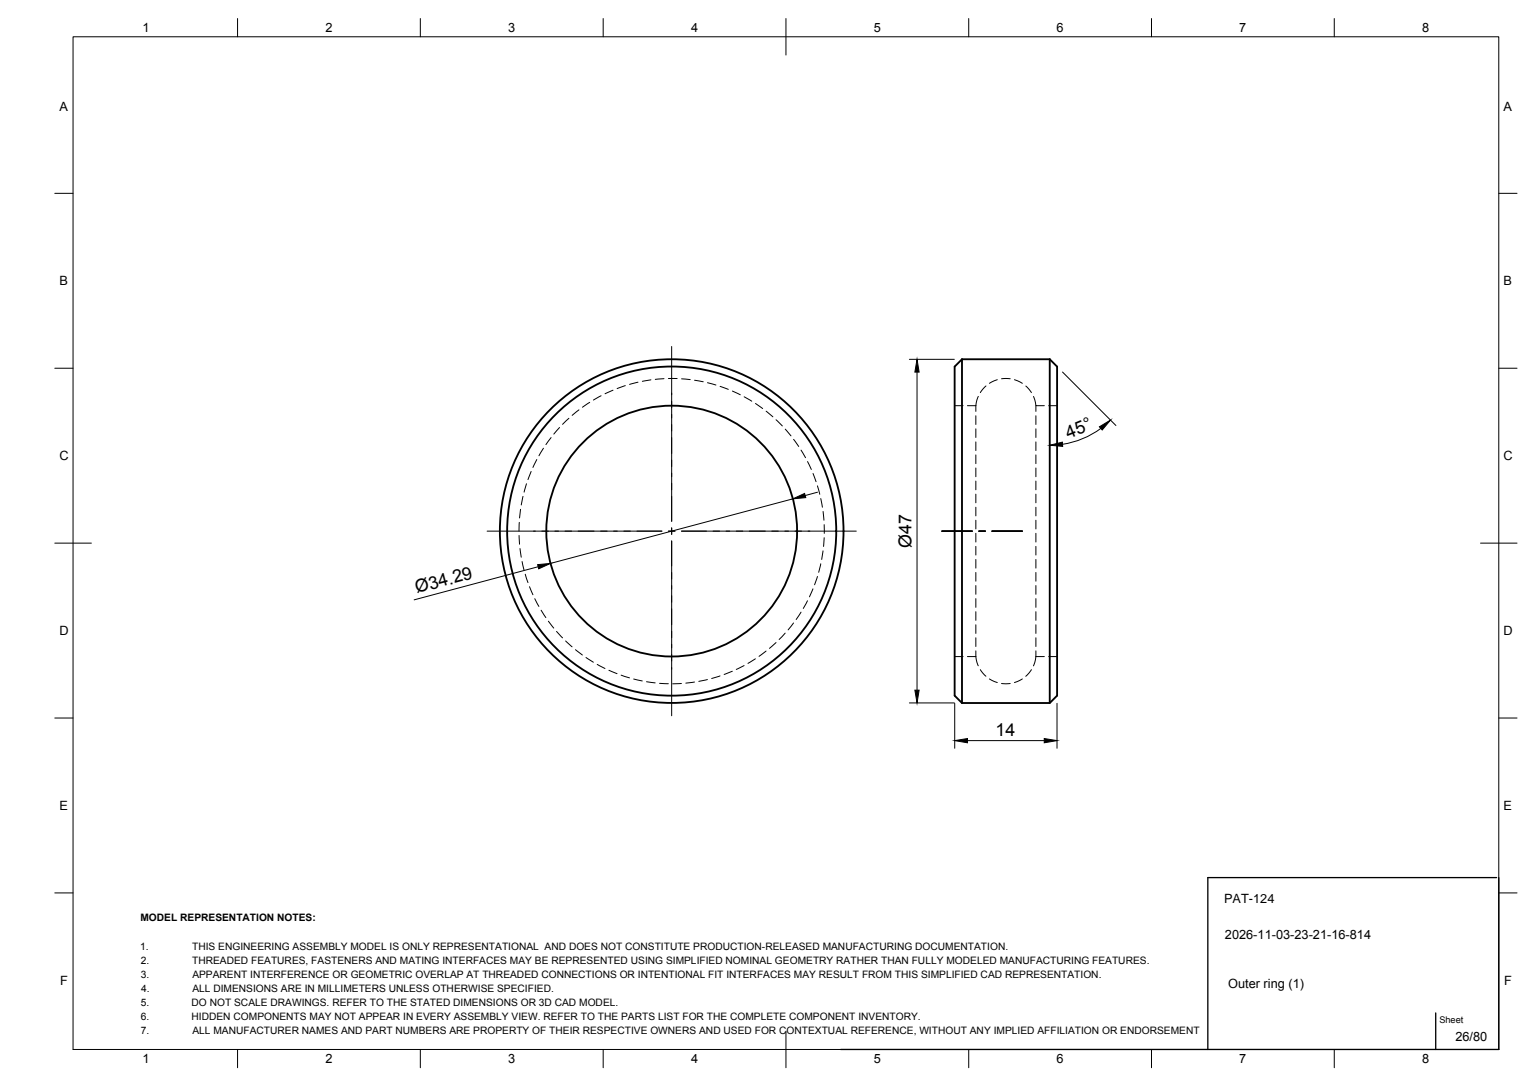
ISO-10303-21;
HEADER;
/* Generated by software containing ST-Developer
 * from STEP Tools, Inc. (www.steptools.com) 
 */

FILE_DESCRIPTION(
/* description */ ('XY cross-slide table'),
/* implementation_level */ '2;1');

FILE_NAME(
/* name */ 'Outer ring (1).step',
/* time_stamp */ '2026-10-28T03:22:46-07:00',
/* author */ (''),
/* organization */ (''),
/* preprocessor_version */ 'ST-DEVELOPER v20.2',
/* originating_system */ 'Autodesk Translation Framework v15.17.0.0',
/* authorisation */ '');

FILE_SCHEMA (('AUTOMOTIVE_DESIGN { 1 0 10303 214 3 1 1 }'));
ENDSEC;

DATA;
#10=MECHANICAL_DESIGN_GEOMETRIC_PRESENTATION_REPRESENTATION('',(#1694),#62984);
#1447=CONICAL_SURFACE('',#24446,2.3,0.785398163397449);
#1448=CONICAL_SURFACE('',#24450,2.3,0.785398163397449);
#1499=TOROIDAL_SURFACE('',#24435,1.675,0.412776);
#1521=SHAPE_REPRESENTATION_RELATIONSHIP('SRR','None',#63371,#1604);
#1604=ADVANCED_BREP_SHAPE_REPRESENTATION('',(#1807),#62908);
#1694=STYLED_ITEM('',(#63912),#1807);
#1807=MANIFOLD_SOLID_BREP('Body1',#22988);
#1994=FACE_BOUND('',#4496,.T.);
#1995=FACE_BOUND('',#4501,.T.);
#2399=PLANE('',#24443);
#2400=PLANE('',#24452);
#3072=FACE_OUTER_BOUND('',#4493,.T.);
#3073=FACE_OUTER_BOUND('',#4494,.T.);
#3074=FACE_OUTER_BOUND('',#4495,.T.);
#3075=FACE_OUTER_BOUND('',#4497,.T.);
#3076=FACE_OUTER_BOUND('',#4498,.T.);
#3077=FACE_OUTER_BOUND('',#4499,.T.);
#3078=FACE_OUTER_BOUND('',#4500,.T.);
#3079=FACE_OUTER_BOUND('',#4502,.T.);
#4493=EDGE_LOOP('',(#15784,#15785,#15786,#15787,#15788,#15789));
#4494=EDGE_LOOP('',(#15790,#15791,#15792,#15793,#15794));
#4495=EDGE_LOOP('',(#15795));
#4496=EDGE_LOOP('',(#15796));
#4497=EDGE_LOOP('',(#15797,#15798,#15799,#15800));
#4498=EDGE_LOOP('',(#15801,#15802,#15803,#15804));
#4499=EDGE_LOOP('',(#15805,#15806,#15807,#15808));
#4500=EDGE_LOOP('',(#15809));
#4501=EDGE_LOOP('',(#15810));
#4502=EDGE_LOOP('',(#15811,#15812,#15813,#15814,#15815));
#6128=LINE('',#34146,#7615);
#6129=LINE('',#34155,#7616);
#6130=LINE('',#34159,#7617);
#6131=LINE('',#34163,#7618);
#6132=LINE('',#34166,#7619);
#7615=VECTOR('',#27569,1.71469);
#7616=VECTOR('',#27580,2.3);
#7617=VECTOR('',#27585,2.35);
#7618=VECTOR('',#27590,2.3);
#7619=VECTOR('',#27595,1.71469);
#9084=CIRCLE('',#24436,1.71469);
#9085=CIRCLE('',#24437,1.71469);
#9086=CIRCLE('',#24438,0.412776);
#9087=CIRCLE('',#24439,1.71469);
#9088=CIRCLE('',#24440,1.71469);
#9089=CIRCLE('',#24442,1.71469);
#9090=CIRCLE('',#24444,2.25);
#9091=CIRCLE('',#24445,1.71469);
#9092=CIRCLE('',#24447,2.35);
#9093=CIRCLE('',#24449,2.35);
#9094=CIRCLE('',#24451,2.25);
#10071=VERTEX_POINT('',#34134);
#10072=VERTEX_POINT('',#34135);
#10073=VERTEX_POINT('',#34138);
#10074=VERTEX_POINT('',#34140);
#10075=VERTEX_POINT('',#34144);
#10076=VERTEX_POINT('',#34148);
#10077=VERTEX_POINT('',#34150);
#10078=VERTEX_POINT('',#34153);
#10079=VERTEX_POINT('',#34157);
#10080=VERTEX_POINT('',#34161);
#12276=EDGE_CURVE('',#10071,#10072,#9084,.T.);
#12277=EDGE_CURVE('',#10072,#10071,#9085,.T.);
#12278=EDGE_CURVE('',#10072,#10073,#9086,.T.);
#12279=EDGE_CURVE('',#10074,#10073,#9087,.T.);
#12280=EDGE_CURVE('',#10073,#10074,#9088,.T.);
#12281=EDGE_CURVE('',#10075,#10075,#9089,.T.);
#12282=EDGE_CURVE('',#10075,#10074,#6128,.T.);
#12283=EDGE_CURVE('',#10076,#10076,#9090,.T.);
#12284=EDGE_CURVE('',#10077,#10077,#9091,.T.);
#12285=EDGE_CURVE('',#10078,#10078,#9092,.T.);
#12286=EDGE_CURVE('',#10078,#10076,#6129,.T.);
#12287=EDGE_CURVE('',#10079,#10079,#9093,.T.);
#12288=EDGE_CURVE('',#10079,#10078,#6130,.T.);
#12289=EDGE_CURVE('',#10080,#10080,#9094,.T.);
#12290=EDGE_CURVE('',#10080,#10079,#6131,.T.);
#12291=EDGE_CURVE('',#10071,#10077,#6132,.T.);
#15784=ORIENTED_EDGE('',*,*,#12276,.F.);
#15785=ORIENTED_EDGE('',*,*,#12277,.F.);
#15786=ORIENTED_EDGE('',*,*,#12278,.T.);
#15787=ORIENTED_EDGE('',*,*,#12279,.F.);
#15788=ORIENTED_EDGE('',*,*,#12280,.F.);
#15789=ORIENTED_EDGE('',*,*,#12278,.F.);
#15790=ORIENTED_EDGE('',*,*,#12281,.T.);
#15791=ORIENTED_EDGE('',*,*,#12282,.T.);
#15792=ORIENTED_EDGE('',*,*,#12279,.T.);
#15793=ORIENTED_EDGE('',*,*,#12280,.T.);
#15794=ORIENTED_EDGE('',*,*,#12282,.F.);
#15795=ORIENTED_EDGE('',*,*,#12283,.F.);
#15796=ORIENTED_EDGE('',*,*,#12284,.T.);
#15797=ORIENTED_EDGE('',*,*,#12285,.F.);
#15798=ORIENTED_EDGE('',*,*,#12286,.T.);
#15799=ORIENTED_EDGE('',*,*,#12283,.T.);
#15800=ORIENTED_EDGE('',*,*,#12286,.F.);
#15801=ORIENTED_EDGE('',*,*,#12287,.F.);
#15802=ORIENTED_EDGE('',*,*,#12288,.T.);
#15803=ORIENTED_EDGE('',*,*,#12285,.T.);
#15804=ORIENTED_EDGE('',*,*,#12288,.F.);
#15805=ORIENTED_EDGE('',*,*,#12289,.F.);
#15806=ORIENTED_EDGE('',*,*,#12290,.T.);
#15807=ORIENTED_EDGE('',*,*,#12287,.T.);
#15808=ORIENTED_EDGE('',*,*,#12290,.F.);
#15809=ORIENTED_EDGE('',*,*,#12289,.T.);
#15810=ORIENTED_EDGE('',*,*,#12281,.F.);
#15811=ORIENTED_EDGE('',*,*,#12276,.T.);
#15812=ORIENTED_EDGE('',*,*,#12277,.T.);
#15813=ORIENTED_EDGE('',*,*,#12291,.T.);
#15814=ORIENTED_EDGE('',*,*,#12284,.F.);
#15815=ORIENTED_EDGE('',*,*,#12291,.F.);
#21117=CYLINDRICAL_SURFACE('',#24441,1.71469);
#21118=CYLINDRICAL_SURFACE('',#24448,2.35);
#21119=CYLINDRICAL_SURFACE('',#24453,1.71469);
#21853=ADVANCED_FACE('',(#3072),#1499,.F.);
#21854=ADVANCED_FACE('',(#3073),#21117,.F.);
#21855=ADVANCED_FACE('',(#3074,#1994),#2399,.T.);
#21856=ADVANCED_FACE('',(#3075),#1447,.T.);
#21857=ADVANCED_FACE('',(#3076),#21118,.T.);
#21858=ADVANCED_FACE('',(#3077),#1448,.T.);
#21859=ADVANCED_FACE('',(#3078,#1995),#2400,.T.);
#21860=ADVANCED_FACE('',(#3079),#21119,.F.);
#22988=CLOSED_SHELL('',(#21853,#21854,#21855,#21856,#21857,#21858,#21859,
#21860));
#24434=AXIS2_PLACEMENT_3D('',#34132,#27551,#27552);
#24435=AXIS2_PLACEMENT_3D('',#34133,#27553,#27554);
#24436=AXIS2_PLACEMENT_3D('',#34136,#27555,#27556);
#24437=AXIS2_PLACEMENT_3D('',#34137,#27557,#27558);
#24438=AXIS2_PLACEMENT_3D('',#34139,#27559,#27560);
#24439=AXIS2_PLACEMENT_3D('',#34141,#27561,#27562);
#24440=AXIS2_PLACEMENT_3D('',#34142,#27563,#27564);
#24441=AXIS2_PLACEMENT_3D('',#34143,#27565,#27566);
#24442=AXIS2_PLACEMENT_3D('',#34145,#27567,#27568);
#24443=AXIS2_PLACEMENT_3D('',#34147,#27570,#27571);
#24444=AXIS2_PLACEMENT_3D('',#34149,#27572,#27573);
#24445=AXIS2_PLACEMENT_3D('',#34151,#27574,#27575);
#24446=AXIS2_PLACEMENT_3D('',#34152,#27576,#27577);
#24447=AXIS2_PLACEMENT_3D('',#34154,#27578,#27579);
#24448=AXIS2_PLACEMENT_3D('',#34156,#27581,#27582);
#24449=AXIS2_PLACEMENT_3D('',#34158,#27583,#27584);
#24450=AXIS2_PLACEMENT_3D('',#34160,#27586,#27587);
#24451=AXIS2_PLACEMENT_3D('',#34162,#27588,#27589);
#24452=AXIS2_PLACEMENT_3D('',#34164,#27591,#27592);
#24453=AXIS2_PLACEMENT_3D('',#34165,#27593,#27594);
#27551=DIRECTION('axis',(0.,0.,1.));
#27552=DIRECTION('refdir',(1.,0.,0.));
#27553=DIRECTION('center_axis',(0.,-1.,0.));
#27554=DIRECTION('ref_axis',(0.,0.,-1.));
#27555=DIRECTION('center_axis',(0.,-1.,0.));
#27556=DIRECTION('ref_axis',(1.,0.,0.));
#27557=DIRECTION('center_axis',(0.,-1.,0.));
#27558=DIRECTION('ref_axis',(1.,0.,0.));
#27559=DIRECTION('center_axis',(1.,0.,1.22464679914735E-16));
#27560=DIRECTION('ref_axis',(-1.22464679914735E-16,0.,1.));
#27561=DIRECTION('center_axis',(0.,1.,0.));
#27562=DIRECTION('ref_axis',(1.,0.,0.));
#27563=DIRECTION('center_axis',(0.,1.,0.));
#27564=DIRECTION('ref_axis',(1.,0.,0.));
#27565=DIRECTION('center_axis',(0.,-1.,0.));
#27566=DIRECTION('ref_axis',(1.,0.,0.));
#27567=DIRECTION('center_axis',(0.,-1.,0.));
#27568=DIRECTION('ref_axis',(1.,0.,0.));
#27569=DIRECTION('',(0.,1.,0.));
#27570=DIRECTION('center_axis',(0.,1.,0.));
#27571=DIRECTION('ref_axis',(0.,0.,1.));
#27572=DIRECTION('center_axis',(0.,-1.,0.));
#27573=DIRECTION('ref_axis',(1.,0.,0.));
#27574=DIRECTION('center_axis',(0.,-1.,0.));
#27575=DIRECTION('ref_axis',(1.,0.,0.));
#27576=DIRECTION('center_axis',(0.,-1.,0.));
#27577=DIRECTION('ref_axis',(1.,0.,0.));
#27578=DIRECTION('center_axis',(0.,-1.,0.));
#27579=DIRECTION('ref_axis',(1.,0.,0.));
#27580=DIRECTION('',(0.707106781186548,0.707106781186547,8.65956056235494E-17));
#27581=DIRECTION('center_axis',(0.,-1.,0.));
#27582=DIRECTION('ref_axis',(1.,0.,0.));
#27583=DIRECTION('center_axis',(0.,-1.,0.));
#27584=DIRECTION('ref_axis',(1.,0.,0.));
#27585=DIRECTION('',(0.,1.,0.));
#27586=DIRECTION('center_axis',(0.,1.,0.));
#27587=DIRECTION('ref_axis',(1.,0.,0.));
#27588=DIRECTION('center_axis',(0.,-1.,0.));
#27589=DIRECTION('ref_axis',(1.,0.,0.));
#27590=DIRECTION('',(-0.707106781186548,0.707106781186547,-8.65956056235494E-17));
#27591=DIRECTION('center_axis',(0.,-1.,0.));
#27592=DIRECTION('ref_axis',(0.,0.,-1.));
#27593=DIRECTION('center_axis',(0.,-1.,0.));
#27594=DIRECTION('ref_axis',(1.,0.,0.));
#27595=DIRECTION('',(0.,1.,0.));
#34132=CARTESIAN_POINT('',(0.,0.,0.));
#34133=CARTESIAN_POINT('Origin',(0.,0.,0.));
#34134=CARTESIAN_POINT('',(-1.71469,0.410863395882378,-2.09988962002998E-16));
#34135=CARTESIAN_POINT('',(-2.09988962002998E-16,0.410863395882378,1.71469));
#34136=CARTESIAN_POINT('Origin',(0.,0.410863395882378,0.));
#34137=CARTESIAN_POINT('Origin',(0.,0.410863395882378,0.));
#34138=CARTESIAN_POINT('',(-2.09988962002998E-16,-0.410863395882378,1.71469));
#34139=CARTESIAN_POINT('Origin',(-2.05128338857182E-16,0.,1.675));
#34140=CARTESIAN_POINT('',(-1.71469,-0.410863395882378,2.09988962002998E-16));
#34141=CARTESIAN_POINT('Origin',(0.,-0.410863395882378,0.));
#34142=CARTESIAN_POINT('Origin',(0.,-0.410863395882378,0.));
#34143=CARTESIAN_POINT('Origin',(0.,0.,0.));
#34144=CARTESIAN_POINT('',(-1.71469,-0.7,-2.09988962002998E-16));
#34145=CARTESIAN_POINT('Origin',(0.,-0.7,0.));
#34146=CARTESIAN_POINT('',(-1.71469,0.,-2.09988962002998E-16));
#34147=CARTESIAN_POINT('Origin',(2.25,0.7,0.));
#34148=CARTESIAN_POINT('',(-2.25,0.7,-2.75545529808154E-16));
#34149=CARTESIAN_POINT('Origin',(0.,0.7,0.));
#34150=CARTESIAN_POINT('',(-1.71469,0.7,-2.09988962002998E-16));
#34151=CARTESIAN_POINT('Origin',(0.,0.7,0.));
#34152=CARTESIAN_POINT('Origin',(0.,0.65,0.));
#34153=CARTESIAN_POINT('',(-2.35,0.6,-2.87791997799628E-16));
#34154=CARTESIAN_POINT('Origin',(0.,0.6,0.));
#34155=CARTESIAN_POINT('',(-2.3,0.65,-2.81668763803891E-16));
#34156=CARTESIAN_POINT('Origin',(0.,0.,0.));
#34157=CARTESIAN_POINT('',(-2.35,-0.6,-2.87791997799628E-16));
#34158=CARTESIAN_POINT('Origin',(0.,-0.6,0.));
#34159=CARTESIAN_POINT('',(-2.35,0.,-2.87791997799628E-16));
#34160=CARTESIAN_POINT('Origin',(0.,-0.65,0.));
#34161=CARTESIAN_POINT('',(-2.25,-0.7,-2.75545529808154E-16));
#34162=CARTESIAN_POINT('Origin',(0.,-0.7,0.));
#34163=CARTESIAN_POINT('',(-2.3,-0.65,-2.81668763803891E-16));
#34164=CARTESIAN_POINT('Origin',(1.71469,-0.7,0.));
#34165=CARTESIAN_POINT('Origin',(0.,0.,0.));
#34166=CARTESIAN_POINT('',(-1.71469,0.,-2.09988962002998E-16));
#62809=UNCERTAINTY_MEASURE_WITH_UNIT(LENGTH_MEASURE(0.001),#62985,
'DISTANCE_ACCURACY_VALUE',
'Maximum model space distance between geometric entities at asserted c
onnectivities');
#62885=UNCERTAINTY_MEASURE_WITH_UNIT(LENGTH_MEASURE(0.001),#62985,
'DISTANCE_ACCURACY_VALUE',
'Maximum model space distance between geometric entities at asserted c
onnectivities');
#62908=(
GEOMETRIC_REPRESENTATION_CONTEXT(3)
GLOBAL_UNCERTAINTY_ASSIGNED_CONTEXT((#62809))
GLOBAL_UNIT_ASSIGNED_CONTEXT((#62985,#62987,#62988))
REPRESENTATION_CONTEXT('','3D')
);
#62984=(
GEOMETRIC_REPRESENTATION_CONTEXT(3)
GLOBAL_UNCERTAINTY_ASSIGNED_CONTEXT((#62885))
GLOBAL_UNIT_ASSIGNED_CONTEXT((#62985,#62987,#62988))
REPRESENTATION_CONTEXT('','3D')
);
#62985=(
LENGTH_UNIT()
NAMED_UNIT(*)
SI_UNIT(.CENTI.,.METRE.)
);
#62987=(
NAMED_UNIT(*)
PLANE_ANGLE_UNIT()
SI_UNIT($,.RADIAN.)
);
#62988=(
NAMED_UNIT(*)
SI_UNIT($,.STERADIAN.)
SOLID_ANGLE_UNIT()
);
#63011=SHAPE_DEFINITION_REPRESENTATION(#63114,#63371);
#63114=PRODUCT_DEFINITION_SHAPE('',$,#63470);
#63371=SHAPE_REPRESENTATION('',(#24434),#62908);
#63447=PRODUCT_DEFINITION_CONTEXT('part definition',#63743,'design');
#63470=PRODUCT_DEFINITION('Outer ring (1)','Outer ring (1)',#63568,#63447);
#63568=PRODUCT_DEFINITION_FORMATION('',$,#63767);
#63743=APPLICATION_CONTEXT(
'Core Data for Automotive Mechanical Design Process');
#63744=PRODUCT_CONTEXT('part definition',#63743,'mechanical');
#63767=PRODUCT('Outer ring (1)','Outer ring (1)','Outer ring (1)',(#63744));
#63906=COLOUR_RGB('Grey',0.48,0.52,0.57);
#63907=FILL_AREA_STYLE_COLOUR('',#63906);
#63908=FILL_AREA_STYLE('',(#63907));
#63909=SURFACE_STYLE_FILL_AREA(#63908);
#63910=SURFACE_SIDE_STYLE('',(#63909));
#63911=SURFACE_STYLE_USAGE(.BOTH.,#63910);
#63912=PRESENTATION_STYLE_ASSIGNMENT((#63911));
ENDSEC;
END-ISO-10303-21;
